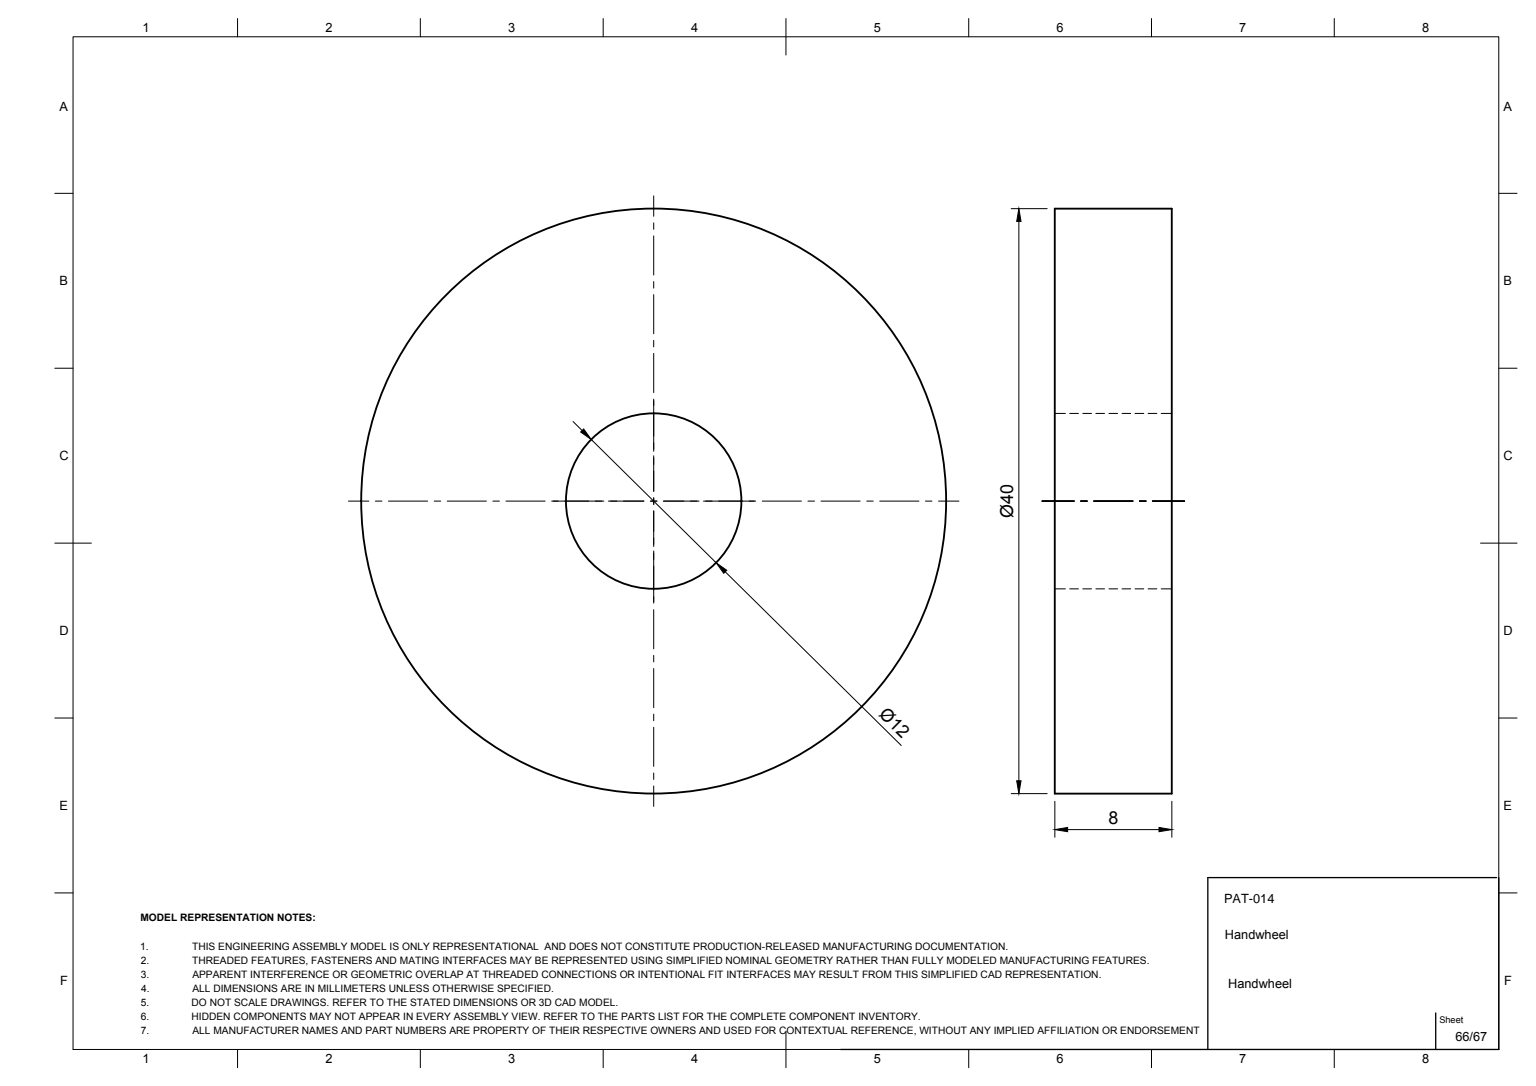
ISO-10303-21;
HEADER;
/* Generated by software containing ST-Developer
 * from STEP Tools, Inc. (www.steptools.com) 
 */

FILE_DESCRIPTION(
/* description */ ('Bin tilter linkage'),
/* implementation_level */ '2;1');

FILE_NAME(
/* name */ 'Handwheel.step',
/* time_stamp */ '2026-10-28T03:26:24-07:00',
/* author */ (''),
/* organization */ (''),
/* preprocessor_version */ 'ST-DEVELOPER v20.2',
/* originating_system */ 'Autodesk Translation Framework v15.17.0.0',
/* authorisation */ '');

FILE_SCHEMA (('AUTOMOTIVE_DESIGN { 1 0 10303 214 3 1 1 }'));
ENDSEC;

DATA;
#10=MECHANICAL_DESIGN_GEOMETRIC_PRESENTATION_REPRESENTATION('',(#974),#23728);
#754=SHAPE_REPRESENTATION_RELATIONSHIP('SRR','None',#24226,#860);
#860=ADVANCED_BREP_SHAPE_REPRESENTATION('',(#1085),#23726);
#974=STYLED_ITEM('',(#24758),#1085);
#1085=MANIFOLD_SOLID_BREP('Body1',#12507);
#1490=FACE_BOUND('',#3843,.T.);
#1491=FACE_BOUND('',#3845,.T.);
#1886=PLANE('',#15454);
#1887=PLANE('',#15455);
#2660=FACE_OUTER_BOUND('',#3840,.T.);
#2661=FACE_OUTER_BOUND('',#3841,.T.);
#2662=FACE_OUTER_BOUND('',#3842,.T.);
#2663=FACE_OUTER_BOUND('',#3844,.T.);
#3840=EDGE_LOOP('',(#11249,#11250,#11251,#11252));
#3841=EDGE_LOOP('',(#11253,#11254,#11255,#11256));
#3842=EDGE_LOOP('',(#11257));
#3843=EDGE_LOOP('',(#11258));
#3844=EDGE_LOOP('',(#11259));
#3845=EDGE_LOOP('',(#11260));
#4521=LINE('',#23464,#5196);
#4522=LINE('',#23470,#5197);
#5196=VECTOR('',#19694,0.6);
#5197=VECTOR('',#19701,2.);
#5951=CIRCLE('',#15449,0.6);
#5952=CIRCLE('',#15450,0.6);
#5953=CIRCLE('',#15452,2.);
#5954=CIRCLE('',#15453,2.);
#6920=VERTEX_POINT('',#23461);
#6921=VERTEX_POINT('',#23463);
#6922=VERTEX_POINT('',#23467);
#6923=VERTEX_POINT('',#23469);
#8364=EDGE_CURVE('',#6920,#6920,#5951,.T.);
#8365=EDGE_CURVE('',#6920,#6921,#4521,.T.);
#8366=EDGE_CURVE('',#6921,#6921,#5952,.T.);
#8367=EDGE_CURVE('',#6922,#6922,#5953,.T.);
#8368=EDGE_CURVE('',#6922,#6923,#4522,.T.);
#8369=EDGE_CURVE('',#6923,#6923,#5954,.T.);
#11249=ORIENTED_EDGE('',*,*,#8364,.F.);
#11250=ORIENTED_EDGE('',*,*,#8365,.T.);
#11251=ORIENTED_EDGE('',*,*,#8366,.T.);
#11252=ORIENTED_EDGE('',*,*,#8365,.F.);
#11253=ORIENTED_EDGE('',*,*,#8367,.F.);
#11254=ORIENTED_EDGE('',*,*,#8368,.T.);
#11255=ORIENTED_EDGE('',*,*,#8369,.T.);
#11256=ORIENTED_EDGE('',*,*,#8368,.F.);
#11257=ORIENTED_EDGE('',*,*,#8367,.T.);
#11258=ORIENTED_EDGE('',*,*,#8364,.T.);
#11259=ORIENTED_EDGE('',*,*,#8369,.F.);
#11260=ORIENTED_EDGE('',*,*,#8366,.F.);
#11612=CYLINDRICAL_SURFACE('',#15448,0.6);
#11613=CYLINDRICAL_SURFACE('',#15451,2.);
#12385=ADVANCED_FACE('',(#2660),#11612,.F.);
#12386=ADVANCED_FACE('',(#2661),#11613,.T.);
#12387=ADVANCED_FACE('',(#2662,#1490),#1886,.T.);
#12388=ADVANCED_FACE('',(#2663,#1491),#1887,.F.);
#12507=CLOSED_SHELL('',(#12385,#12386,#12387,#12388));
#15447=AXIS2_PLACEMENT_3D('',#23459,#19688,#19689);
#15448=AXIS2_PLACEMENT_3D('',#23460,#19690,#19691);
#15449=AXIS2_PLACEMENT_3D('',#23462,#19692,#19693);
#15450=AXIS2_PLACEMENT_3D('',#23465,#19695,#19696);
#15451=AXIS2_PLACEMENT_3D('',#23466,#19697,#19698);
#15452=AXIS2_PLACEMENT_3D('',#23468,#19699,#19700);
#15453=AXIS2_PLACEMENT_3D('',#23471,#19702,#19703);
#15454=AXIS2_PLACEMENT_3D('',#23472,#19704,#19705);
#15455=AXIS2_PLACEMENT_3D('',#23473,#19706,#19707);
#19688=DIRECTION('axis',(0.,0.,1.));
#19689=DIRECTION('refdir',(1.,0.,0.));
#19690=DIRECTION('center_axis',(1.,0.,0.));
#19691=DIRECTION('ref_axis',(0.,0.,-1.));
#19692=DIRECTION('center_axis',(-1.,0.,0.));
#19693=DIRECTION('ref_axis',(0.,0.,-1.));
#19694=DIRECTION('',(-1.,0.,0.));
#19695=DIRECTION('center_axis',(-1.,0.,0.));
#19696=DIRECTION('ref_axis',(0.,0.,-1.));
#19697=DIRECTION('center_axis',(1.,0.,0.));
#19698=DIRECTION('ref_axis',(0.,0.,-1.));
#19699=DIRECTION('center_axis',(1.,0.,0.));
#19700=DIRECTION('ref_axis',(0.,0.,-1.));
#19701=DIRECTION('',(-1.,0.,0.));
#19702=DIRECTION('center_axis',(1.,0.,0.));
#19703=DIRECTION('ref_axis',(0.,0.,-1.));
#19704=DIRECTION('center_axis',(1.,0.,0.));
#19705=DIRECTION('ref_axis',(0.,0.,-1.));
#19706=DIRECTION('center_axis',(1.,0.,0.));
#19707=DIRECTION('ref_axis',(0.,0.,-1.));
#23459=CARTESIAN_POINT('',(0.,0.,0.));
#23460=CARTESIAN_POINT('Origin',(-12.5,-4.5,8.));
#23461=CARTESIAN_POINT('',(-11.7,-4.5,8.6));
#23462=CARTESIAN_POINT('Origin',(-11.7,-4.5,8.));
#23463=CARTESIAN_POINT('',(-12.5,-4.5,8.6));
#23464=CARTESIAN_POINT('',(-12.5,-4.5,8.6));
#23465=CARTESIAN_POINT('Origin',(-12.5,-4.5,8.));
#23466=CARTESIAN_POINT('Origin',(-12.5,-4.5,8.));
#23467=CARTESIAN_POINT('',(-11.7,-4.5,10.));
#23468=CARTESIAN_POINT('Origin',(-11.7,-4.5,8.));
#23469=CARTESIAN_POINT('',(-12.5,-4.5,10.));
#23470=CARTESIAN_POINT('',(-12.5,-4.5,10.));
#23471=CARTESIAN_POINT('Origin',(-12.5,-4.5,8.));
#23472=CARTESIAN_POINT('Origin',(-11.7,-4.5,8.));
#23473=CARTESIAN_POINT('Origin',(-12.5,-4.5,8.));
#23609=UNCERTAINTY_MEASURE_WITH_UNIT(LENGTH_MEASURE(0.001),#23729,
'DISTANCE_ACCURACY_VALUE',
'Maximum model space distance between geometric entities at asserted c
onnectivities');
#23611=UNCERTAINTY_MEASURE_WITH_UNIT(LENGTH_MEASURE(0.001),#23729,
'DISTANCE_ACCURACY_VALUE',
'Maximum model space distance between geometric entities at asserted c
onnectivities');
#23726=(
GEOMETRIC_REPRESENTATION_CONTEXT(3)
GLOBAL_UNCERTAINTY_ASSIGNED_CONTEXT((#23609))
GLOBAL_UNIT_ASSIGNED_CONTEXT((#23729,#23731,#23732))
REPRESENTATION_CONTEXT('','3D')
);
#23728=(
GEOMETRIC_REPRESENTATION_CONTEXT(3)
GLOBAL_UNCERTAINTY_ASSIGNED_CONTEXT((#23611))
GLOBAL_UNIT_ASSIGNED_CONTEXT((#23729,#23731,#23732))
REPRESENTATION_CONTEXT('','3D')
);
#23729=(
LENGTH_UNIT()
NAMED_UNIT(*)
SI_UNIT(.CENTI.,.METRE.)
);
#23731=(
NAMED_UNIT(*)
PLANE_ANGLE_UNIT()
SI_UNIT($,.RADIAN.)
);
#23732=(
NAMED_UNIT(*)
SI_UNIT($,.STERADIAN.)
SOLID_ANGLE_UNIT()
);
#23847=SHAPE_DEFINITION_REPRESENTATION(#24098,#24226);
#24098=PRODUCT_DEFINITION_SHAPE('',$,#24343);
#24226=SHAPE_REPRESENTATION('',(#15447),#23726);
#24228=PRODUCT_DEFINITION_CONTEXT('part definition',#24578,'design');
#24343=PRODUCT_DEFINITION('Handwheel','Handwheel',#24459,#24228);
#24459=PRODUCT_DEFINITION_FORMATION('',$,#24694);
#24578=APPLICATION_CONTEXT(
'Core Data for Automotive Mechanical Design Process');
#24579=PRODUCT_CONTEXT('part definition',#24578,'mechanical');
#24694=PRODUCT('Handwheel','Handwheel','Handwheel',(#24579));
#24752=COLOUR_RGB('Sky Blue',0.24,0.69,0.87);
#24753=FILL_AREA_STYLE_COLOUR('',#24752);
#24754=FILL_AREA_STYLE('',(#24753));
#24755=SURFACE_STYLE_FILL_AREA(#24754);
#24756=SURFACE_SIDE_STYLE('',(#24755));
#24757=SURFACE_STYLE_USAGE(.BOTH.,#24756);
#24758=PRESENTATION_STYLE_ASSIGNMENT((#24757));
ENDSEC;
END-ISO-10303-21;
